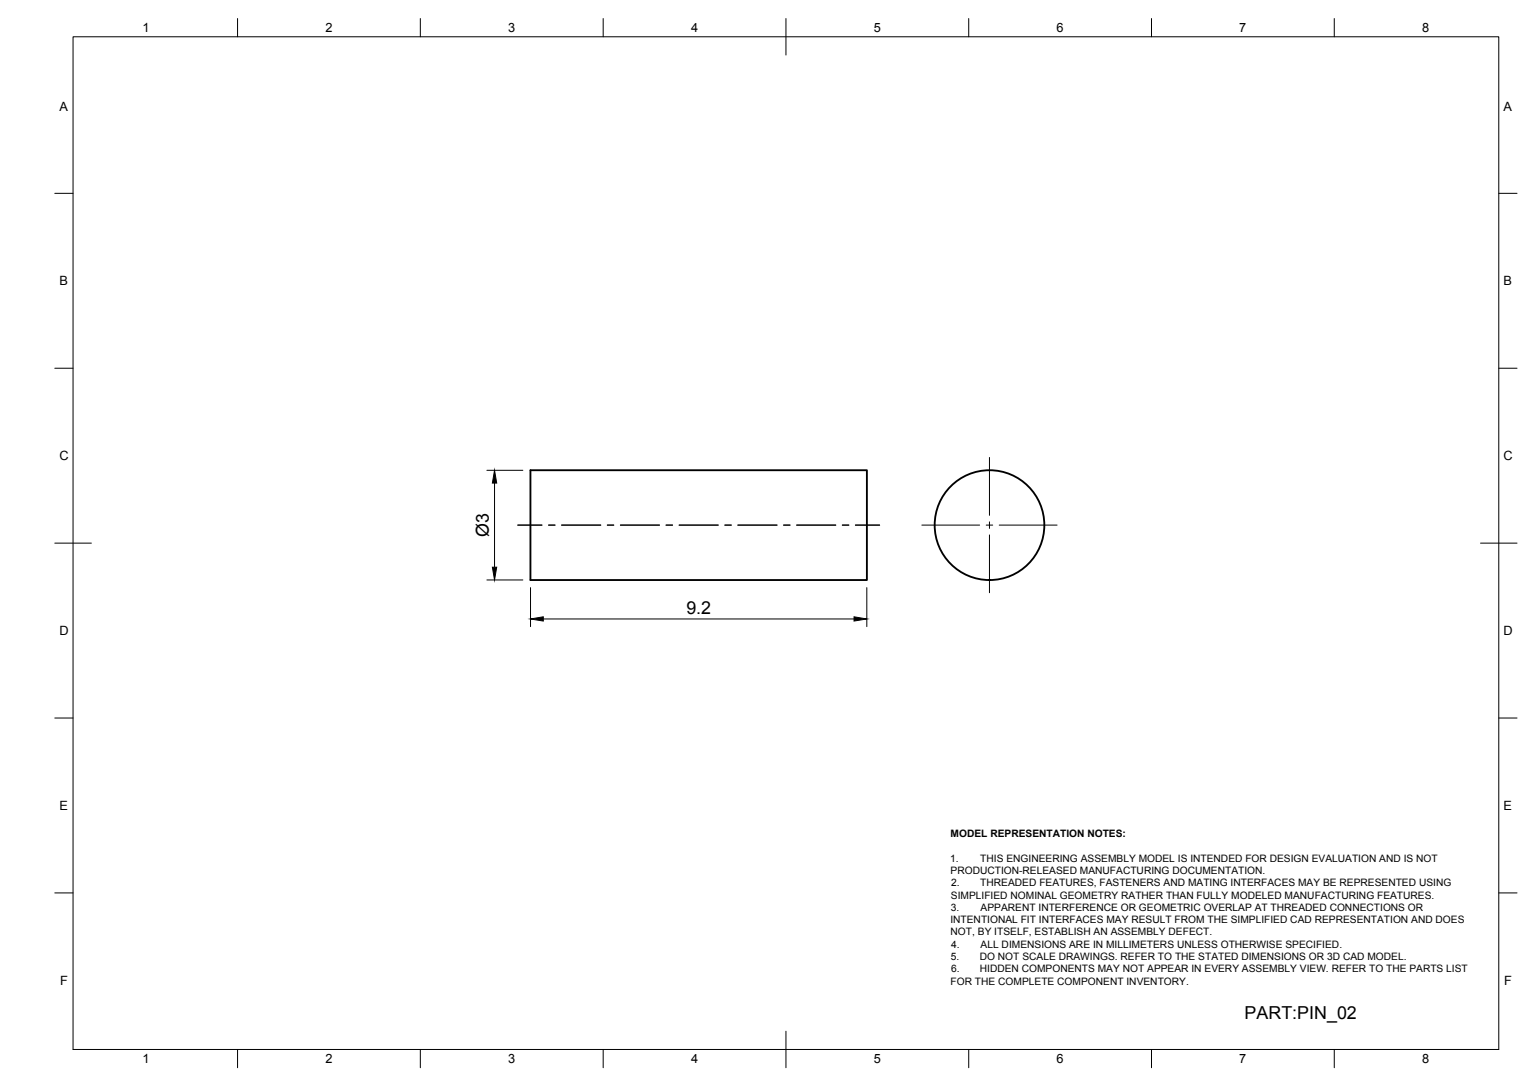
ISO-10303-21;
HEADER;
/* Generated by software containing ST-Developer
 * from STEP Tools, Inc. (www.steptools.com) 
 */

FILE_DESCRIPTION(
/* description */ (''),
/* implementation_level */ '2;1');

FILE_NAME(
/* name */ 'Pin_02.step',
/* time_stamp */ '2026-10-05T13:12:53-07:00',
/* author */ (''),
/* organization */ (''),
/* preprocessor_version */ 'ST-DEVELOPER v20.2',
/* originating_system */ 'Autodesk Translation Framework v15.15.0.0',
/* authorisation */ '');

FILE_SCHEMA (('AUTOMOTIVE_DESIGN { 1 0 10303 214 3 1 1 }'));
ENDSEC;

DATA;
#10=MECHANICAL_DESIGN_GEOMETRIC_PRESENTATION_REPRESENTATION('',(#65),#5912);
#49=SHAPE_REPRESENTATION_RELATIONSHIP('SRR','None',#5950,#57);
#57=ADVANCED_BREP_SHAPE_REPRESENTATION('',(#73),#5910);
#65=STYLED_ITEM('',(#5994),#73);
#73=MANIFOLD_SOLID_BREP('Body1',#3476);
#166=CYLINDRICAL_SURFACE('',#3869,1.4999996247669);
#344=FACE_OUTER_BOUND('',#547,.T.);
#345=FACE_OUTER_BOUND('',#548,.T.);
#346=FACE_OUTER_BOUND('',#549,.T.);
#547=EDGE_LOOP('',(#3148));
#548=EDGE_LOOP('',(#3149,#3150,#3151,#3152));
#549=EDGE_LOOP('',(#3153));
#651=CIRCLE('',#3868,1.4999996247669);
#652=CIRCLE('',#3870,1.4999996247669);
#1018=LINE('',#5874,#1383);
#1383=VECTOR('',#4857,1.4999996247669);
#1701=VERTEX_POINT('',#5869);
#1702=VERTEX_POINT('',#5872);
#2184=EDGE_CURVE('',#1701,#1701,#651,.T.);
#2185=EDGE_CURVE('',#1702,#1702,#652,.T.);
#2186=EDGE_CURVE('',#1702,#1701,#1018,.T.);
#3148=ORIENTED_EDGE('',*,*,#2184,.T.);
#3149=ORIENTED_EDGE('',*,*,#2185,.F.);
#3150=ORIENTED_EDGE('',*,*,#2186,.T.);
#3151=ORIENTED_EDGE('',*,*,#2184,.F.);
#3152=ORIENTED_EDGE('',*,*,#2186,.F.);
#3153=ORIENTED_EDGE('',*,*,#2185,.T.);
#3284=PLANE('',#3867);
#3285=PLANE('',#3871);
#3464=ADVANCED_FACE('',(#344),#3284,.F.);
#3465=ADVANCED_FACE('',(#345),#166,.T.);
#3466=ADVANCED_FACE('',(#346),#3285,.T.);
#3476=CLOSED_SHELL('',(#3464,#3465,#3466));
#3866=AXIS2_PLACEMENT_3D('',#5867,#4847,#4848);
#3867=AXIS2_PLACEMENT_3D('',#5868,#4849,#4850);
#3868=AXIS2_PLACEMENT_3D('',#5870,#4851,#4852);
#3869=AXIS2_PLACEMENT_3D('',#5871,#4853,#4854);
#3870=AXIS2_PLACEMENT_3D('',#5873,#4855,#4856);
#3871=AXIS2_PLACEMENT_3D('',#5875,#4858,#4859);
#4847=DIRECTION('axis',(0.,0.,1.));
#4848=DIRECTION('refdir',(1.,0.,0.));
#4849=DIRECTION('center_axis',(0.,-1.,0.));
#4850=DIRECTION('ref_axis',(1.,0.,0.));
#4851=DIRECTION('center_axis',(0.,1.,0.));
#4852=DIRECTION('ref_axis',(1.,0.,0.));
#4853=DIRECTION('center_axis',(0.,-1.,0.));
#4854=DIRECTION('ref_axis',(1.,0.,0.));
#4855=DIRECTION('center_axis',(0.,-1.,0.));
#4856=DIRECTION('ref_axis',(1.,0.,0.));
#4857=DIRECTION('',(0.,1.,0.));
#4858=DIRECTION('center_axis',(0.,-1.,0.));
#4859=DIRECTION('ref_axis',(1.,0.,0.));
#5867=CARTESIAN_POINT('',(0.,0.,0.));
#5868=CARTESIAN_POINT('Origin',(100.979996788778,-2.8,2.49999516053467));
#5869=CARTESIAN_POINT('',(99.4799971640107,-2.8,2.49999516053467));
#5870=CARTESIAN_POINT('Origin',(100.979996788778,-2.8,2.49999516053467));
#5871=CARTESIAN_POINT('Origin',(100.979996788778,-8.,2.49999516053467));
#5872=CARTESIAN_POINT('',(99.4799971640107,-12.,2.49999516053467));
#5873=CARTESIAN_POINT('Origin',(100.979996788778,-12.,2.49999516053467));
#5874=CARTESIAN_POINT('',(99.4799971640111,-8.,2.49999516053467));
#5875=CARTESIAN_POINT('Origin',(100.979996788778,-12.,2.49999516053467));
#5900=UNCERTAINTY_MEASURE_WITH_UNIT(LENGTH_MEASURE(0.01),#5913,
'DISTANCE_ACCURACY_VALUE',
'Maximum model space distance between geometric entities at asserted c
onnectivities');
#5902=UNCERTAINTY_MEASURE_WITH_UNIT(LENGTH_MEASURE(0.01),#5913,
'DISTANCE_ACCURACY_VALUE',
'Maximum model space distance between geometric entities at asserted c
onnectivities');
#5910=(
GEOMETRIC_REPRESENTATION_CONTEXT(3)
GLOBAL_UNCERTAINTY_ASSIGNED_CONTEXT((#5900))
GLOBAL_UNIT_ASSIGNED_CONTEXT((#5913,#5915,#5916))
REPRESENTATION_CONTEXT('','3D')
);
#5912=(
GEOMETRIC_REPRESENTATION_CONTEXT(3)
GLOBAL_UNCERTAINTY_ASSIGNED_CONTEXT((#5902))
GLOBAL_UNIT_ASSIGNED_CONTEXT((#5913,#5915,#5916))
REPRESENTATION_CONTEXT('','3D')
);
#5913=(
LENGTH_UNIT()
NAMED_UNIT(*)
SI_UNIT(.MILLI.,.METRE.)
);
#5915=(
NAMED_UNIT(*)
PLANE_ANGLE_UNIT()
SI_UNIT($,.RADIAN.)
);
#5916=(
NAMED_UNIT(*)
SI_UNIT($,.STERADIAN.)
SOLID_ANGLE_UNIT()
);
#5924=SHAPE_DEFINITION_REPRESENTATION(#5933,#5950);
#5933=PRODUCT_DEFINITION_SHAPE('',$,#5960);
#5950=SHAPE_REPRESENTATION('',(#3866),#5910);
#5952=PRODUCT_DEFINITION_CONTEXT('part definition',#5981,'design');
#5960=PRODUCT_DEFINITION('Pin_02','Pin_02',#5969,#5952);
#5969=PRODUCT_DEFINITION_FORMATION('',$,#5990);
#5981=APPLICATION_CONTEXT(
'Core Data for Automotive Mechanical Design Process');
#5982=PRODUCT_CONTEXT('part definition',#5981,'mechanical');
#5990=PRODUCT('Pin_02','Pin_02',$,(#5982));
#5994=PRESENTATION_STYLE_ASSIGNMENT((#5997));
#5997=SURFACE_STYLE_USAGE(.BOTH.,#6000);
#6000=SURFACE_SIDE_STYLE('',(#6003));
#6003=SURFACE_STYLE_FILL_AREA(#6006);
#6006=FILL_AREA_STYLE('Opaque(160,160,160)',(#6009));
#6009=FILL_AREA_STYLE_COLOUR('Opaque(160,160,160)',#6012);
#6012=COLOUR_RGB('Opaque(160,160,160)', 0.31764706, 0.68627451, 0.89019608);
ENDSEC;
END-ISO-10303-21;
